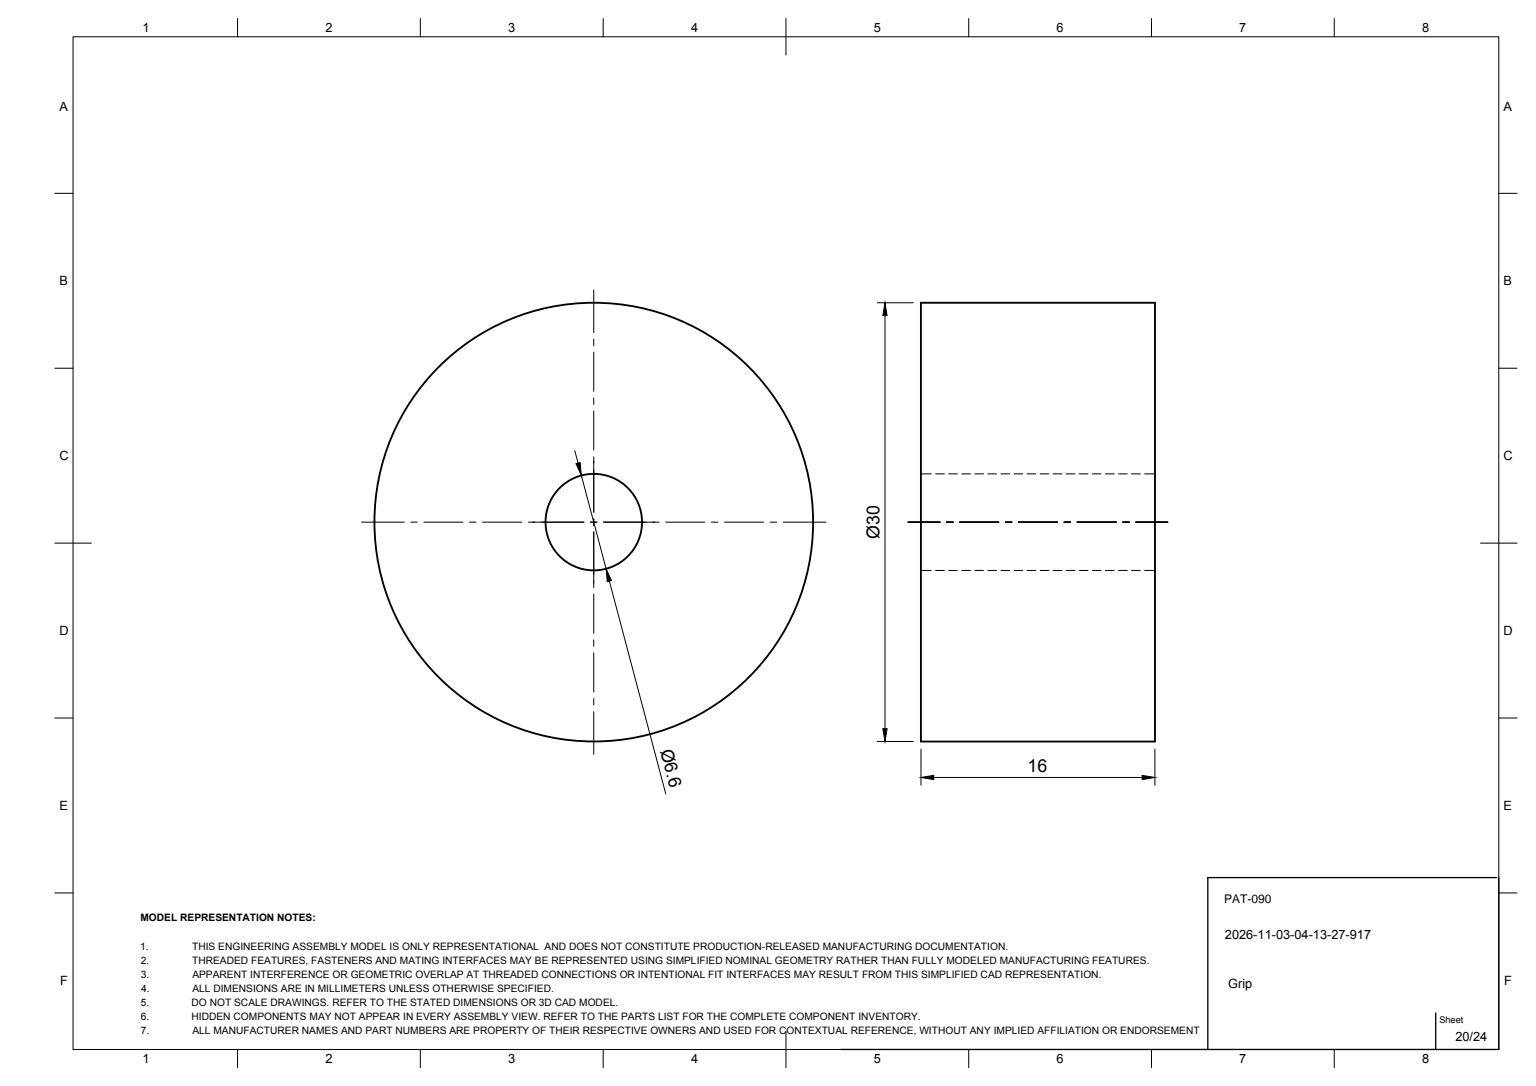
ISO-10303-21;
HEADER;
/* Generated by software containing ST-Developer
 * from STEP Tools, Inc. (www.steptools.com) 
 */

FILE_DESCRIPTION(
/* description */ ('Round-Shaft Linear Stage with Ball Bushings'),
/* implementation_level */ '2;1');

FILE_NAME(
/* name */ 'Grip.step',
/* time_stamp */ '2026-10-27T10:47:55-07:00',
/* author */ (''),
/* organization */ (''),
/* preprocessor_version */ 'ST-DEVELOPER v20.2',
/* originating_system */ 'Autodesk Translation Framework v15.17.0.0',
/* authorisation */ '');

FILE_SCHEMA (('AUTOMOTIVE_DESIGN { 1 0 10303 214 3 1 1 }'));
ENDSEC;

DATA;
#10=MECHANICAL_DESIGN_GEOMETRIC_PRESENTATION_REPRESENTATION('',(#316),#7835);
#274=SHAPE_REPRESENTATION_RELATIONSHIP('SRR','None',#7963,#295);
#295=ADVANCED_BREP_SHAPE_REPRESENTATION('',(#336),#7827);
#316=STYLED_ITEM('',(#8151),#336);
#336=MANIFOLD_SOLID_BREP('Body1',#4407);
#441=FACE_BOUND('',#1150,.T.);
#442=FACE_BOUND('',#1152,.T.);
#562=PLANE('',#4981);
#563=PLANE('',#4982);
#789=FACE_OUTER_BOUND('',#1147,.T.);
#790=FACE_OUTER_BOUND('',#1148,.T.);
#791=FACE_OUTER_BOUND('',#1149,.T.);
#792=FACE_OUTER_BOUND('',#1151,.T.);
#1147=EDGE_LOOP('',(#3740,#3741,#3742,#3743));
#1148=EDGE_LOOP('',(#3744,#3745,#3746,#3747));
#1149=EDGE_LOOP('',(#3748));
#1150=EDGE_LOOP('',(#3749));
#1151=EDGE_LOOP('',(#3750));
#1152=EDGE_LOOP('',(#3751));
#1487=LINE('',#7385,#1827);
#1488=LINE('',#7391,#1828);
#1827=VECTOR('',#6070,0.33);
#1828=VECTOR('',#6077,1.5);
#2064=CIRCLE('',#4976,0.33);
#2065=CIRCLE('',#4977,0.33);
#2066=CIRCLE('',#4979,1.5);
#2067=CIRCLE('',#4980,1.5);
#2365=VERTEX_POINT('',#7382);
#2366=VERTEX_POINT('',#7384);
#2367=VERTEX_POINT('',#7388);
#2368=VERTEX_POINT('',#7390);
#2838=EDGE_CURVE('',#2365,#2365,#2064,.T.);
#2839=EDGE_CURVE('',#2365,#2366,#1487,.T.);
#2840=EDGE_CURVE('',#2366,#2366,#2065,.T.);
#2841=EDGE_CURVE('',#2367,#2367,#2066,.T.);
#2842=EDGE_CURVE('',#2367,#2368,#1488,.T.);
#2843=EDGE_CURVE('',#2368,#2368,#2067,.T.);
#3740=ORIENTED_EDGE('',*,*,#2838,.F.);
#3741=ORIENTED_EDGE('',*,*,#2839,.T.);
#3742=ORIENTED_EDGE('',*,*,#2840,.T.);
#3743=ORIENTED_EDGE('',*,*,#2839,.F.);
#3744=ORIENTED_EDGE('',*,*,#2841,.F.);
#3745=ORIENTED_EDGE('',*,*,#2842,.T.);
#3746=ORIENTED_EDGE('',*,*,#2843,.T.);
#3747=ORIENTED_EDGE('',*,*,#2842,.F.);
#3748=ORIENTED_EDGE('',*,*,#2841,.T.);
#3749=ORIENTED_EDGE('',*,*,#2838,.T.);
#3750=ORIENTED_EDGE('',*,*,#2843,.F.);
#3751=ORIENTED_EDGE('',*,*,#2840,.F.);
#4117=CYLINDRICAL_SURFACE('',#4975,0.33);
#4118=CYLINDRICAL_SURFACE('',#4978,1.5);
#4308=ADVANCED_FACE('',(#789),#4117,.F.);
#4309=ADVANCED_FACE('',(#790),#4118,.T.);
#4310=ADVANCED_FACE('',(#791,#441),#562,.T.);
#4311=ADVANCED_FACE('',(#792,#442),#563,.F.);
#4407=CLOSED_SHELL('',(#4308,#4309,#4310,#4311));
#4974=AXIS2_PLACEMENT_3D('',#7380,#6064,#6065);
#4975=AXIS2_PLACEMENT_3D('',#7381,#6066,#6067);
#4976=AXIS2_PLACEMENT_3D('',#7383,#6068,#6069);
#4977=AXIS2_PLACEMENT_3D('',#7386,#6071,#6072);
#4978=AXIS2_PLACEMENT_3D('',#7387,#6073,#6074);
#4979=AXIS2_PLACEMENT_3D('',#7389,#6075,#6076);
#4980=AXIS2_PLACEMENT_3D('',#7392,#6078,#6079);
#4981=AXIS2_PLACEMENT_3D('',#7393,#6080,#6081);
#4982=AXIS2_PLACEMENT_3D('',#7394,#6082,#6083);
#6064=DIRECTION('axis',(0.,0.,1.));
#6065=DIRECTION('refdir',(1.,0.,0.));
#6066=DIRECTION('center_axis',(0.,0.,1.));
#6067=DIRECTION('ref_axis',(1.,0.,0.));
#6068=DIRECTION('center_axis',(0.,0.,-1.));
#6069=DIRECTION('ref_axis',(1.,0.,0.));
#6070=DIRECTION('',(0.,0.,-1.));
#6071=DIRECTION('center_axis',(0.,0.,-1.));
#6072=DIRECTION('ref_axis',(1.,0.,0.));
#6073=DIRECTION('center_axis',(0.,0.,1.));
#6074=DIRECTION('ref_axis',(1.,0.,0.));
#6075=DIRECTION('center_axis',(0.,0.,1.));
#6076=DIRECTION('ref_axis',(1.,0.,0.));
#6077=DIRECTION('',(0.,0.,-1.));
#6078=DIRECTION('center_axis',(0.,0.,1.));
#6079=DIRECTION('ref_axis',(1.,0.,0.));
#6080=DIRECTION('center_axis',(0.,0.,1.));
#6081=DIRECTION('ref_axis',(1.,0.,0.));
#6082=DIRECTION('center_axis',(0.,0.,1.));
#6083=DIRECTION('ref_axis',(1.,0.,0.));
#7380=CARTESIAN_POINT('',(0.,0.,0.));
#7381=CARTESIAN_POINT('Origin',(15.,0.,6.6));
#7382=CARTESIAN_POINT('',(14.67,-4.04133443718627E-17,8.2));
#7383=CARTESIAN_POINT('Origin',(15.,0.,8.2));
#7384=CARTESIAN_POINT('',(14.67,-4.04133443718627E-17,6.6));
#7385=CARTESIAN_POINT('',(14.67,-4.04133443718627E-17,6.6));
#7386=CARTESIAN_POINT('Origin',(15.,0.,6.6));
#7387=CARTESIAN_POINT('Origin',(15.,0.,6.6));
#7388=CARTESIAN_POINT('',(13.5,-1.83697019872103E-16,8.2));
#7389=CARTESIAN_POINT('Origin',(15.,0.,8.2));
#7390=CARTESIAN_POINT('',(13.5,-1.83697019872103E-16,6.6));
#7391=CARTESIAN_POINT('',(13.5,-1.83697019872103E-16,6.6));
#7392=CARTESIAN_POINT('Origin',(15.,0.,6.6));
#7393=CARTESIAN_POINT('Origin',(15.,0.,8.2));
#7394=CARTESIAN_POINT('Origin',(15.,0.,6.6));
#7801=UNCERTAINTY_MEASURE_WITH_UNIT(LENGTH_MEASURE(0.001),#7836,
'DISTANCE_ACCURACY_VALUE',
'Maximum model space distance between geometric entities at asserted c
onnectivities');
#7809=UNCERTAINTY_MEASURE_WITH_UNIT(LENGTH_MEASURE(0.001),#7836,
'DISTANCE_ACCURACY_VALUE',
'Maximum model space distance between geometric entities at asserted c
onnectivities');
#7827=(
GEOMETRIC_REPRESENTATION_CONTEXT(3)
GLOBAL_UNCERTAINTY_ASSIGNED_CONTEXT((#7801))
GLOBAL_UNIT_ASSIGNED_CONTEXT((#7836,#7838,#7839))
REPRESENTATION_CONTEXT('','3D')
);
#7835=(
GEOMETRIC_REPRESENTATION_CONTEXT(3)
GLOBAL_UNCERTAINTY_ASSIGNED_CONTEXT((#7809))
GLOBAL_UNIT_ASSIGNED_CONTEXT((#7836,#7838,#7839))
REPRESENTATION_CONTEXT('','3D')
);
#7836=(
LENGTH_UNIT()
NAMED_UNIT(*)
SI_UNIT(.CENTI.,.METRE.)
);
#7838=(
NAMED_UNIT(*)
PLANE_ANGLE_UNIT()
SI_UNIT($,.RADIAN.)
);
#7839=(
NAMED_UNIT(*)
SI_UNIT($,.STERADIAN.)
SOLID_ANGLE_UNIT()
);
#7857=SHAPE_DEFINITION_REPRESENTATION(#7882,#7963);
#7882=PRODUCT_DEFINITION_SHAPE('',$,#7989);
#7963=SHAPE_REPRESENTATION('',(#4974),#7827);
#7971=PRODUCT_DEFINITION_CONTEXT('part definition',#8048,'design');
#7989=PRODUCT_DEFINITION('Grip','Grip',#8014,#7971);
#8014=PRODUCT_DEFINITION_FORMATION('',$,#8067);
#8048=APPLICATION_CONTEXT(
'Core Data for Automotive Mechanical Design Process');
#8049=PRODUCT_CONTEXT('part definition',#8048,'mechanical');
#8067=PRODUCT('Grip','Grip','Grip',(#8049));
#8145=COLOUR_RGB('Black',0.12,0.14,0.17);
#8146=FILL_AREA_STYLE_COLOUR('',#8145);
#8147=FILL_AREA_STYLE('',(#8146));
#8148=SURFACE_STYLE_FILL_AREA(#8147);
#8149=SURFACE_SIDE_STYLE('',(#8148));
#8150=SURFACE_STYLE_USAGE(.BOTH.,#8149);
#8151=PRESENTATION_STYLE_ASSIGNMENT((#8150));
ENDSEC;
END-ISO-10303-21;
